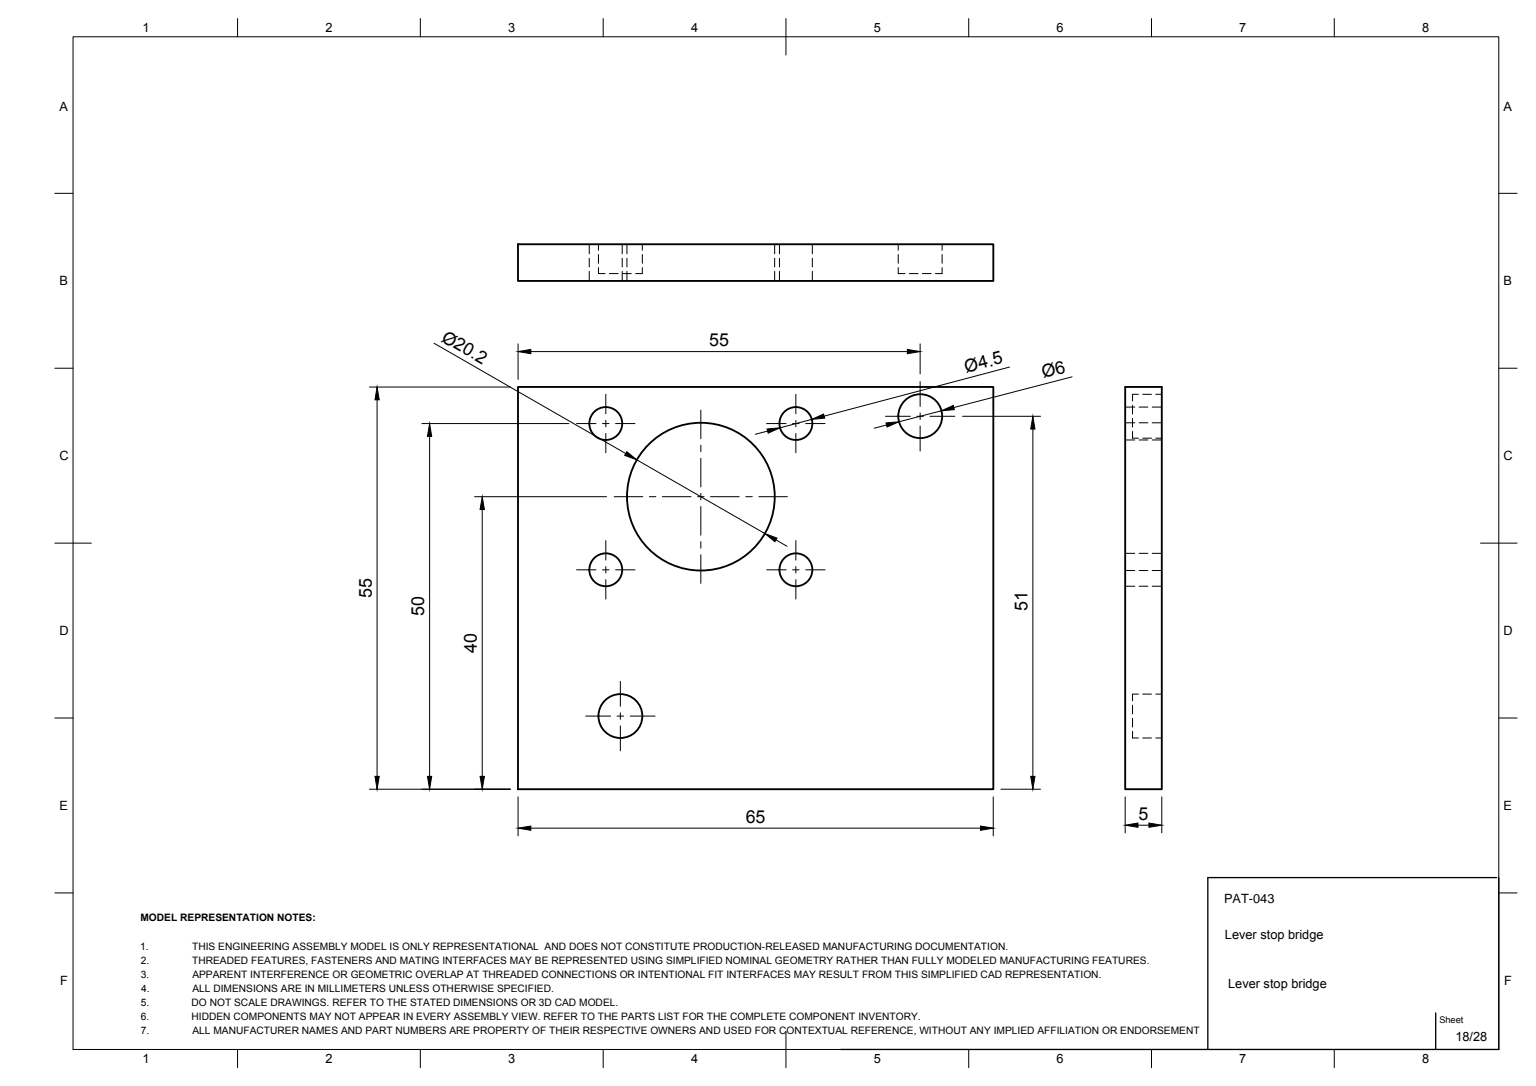
ISO-10303-21;
HEADER;
/* Generated by software containing ST-Developer
 * from STEP Tools, Inc. (www.steptools.com) 
 */

FILE_DESCRIPTION(
/* description */ ('Four-valve pipe header'),
/* implementation_level */ '2;1');

FILE_NAME(
/* name */ 'Lever stop bridge.step',
/* time_stamp */ '2026-10-29T16:56:19-07:00',
/* author */ (''),
/* organization */ (''),
/* preprocessor_version */ 'ST-DEVELOPER v20.2',
/* originating_system */ 'Autodesk Translation Framework v15.17.0.0',
/* authorisation */ '');

FILE_SCHEMA (('AUTOMOTIVE_DESIGN { 1 0 10303 214 3 1 1 }'));
ENDSEC;

DATA;
#10=MECHANICAL_DESIGN_GEOMETRIC_PRESENTATION_REPRESENTATION('',(#344),#10119);
#292=SHAPE_REPRESENTATION_RELATIONSHIP('SRR','None',#10254,#318);
#318=ADVANCED_BREP_SHAPE_REPRESENTATION('',(#370),#10103);
#344=STYLED_ITEM('',(#10456),#370);
#370=MANIFOLD_SOLID_BREP('Body1',#5590);
#498=FACE_BOUND('',#1339,.T.);
#499=FACE_BOUND('',#1340,.T.);
#500=FACE_BOUND('',#1341,.T.);
#501=FACE_BOUND('',#1342,.T.);
#502=FACE_BOUND('',#1343,.T.);
#503=FACE_BOUND('',#1344,.T.);
#504=FACE_BOUND('',#1345,.T.);
#505=FACE_BOUND('',#1347,.T.);
#506=FACE_BOUND('',#1348,.T.);
#507=FACE_BOUND('',#1349,.T.);
#508=FACE_BOUND('',#1350,.T.);
#509=FACE_BOUND('',#1351,.T.);
#636=PLANE('',#6253);
#637=PLANE('',#6257);
#638=PLANE('',#6273);
#639=PLANE('',#6274);
#640=PLANE('',#6275);
#641=PLANE('',#6276);
#642=PLANE('',#6277);
#643=PLANE('',#6278);
#921=FACE_OUTER_BOUND('',#1325,.T.);
#922=FACE_OUTER_BOUND('',#1326,.T.);
#923=FACE_OUTER_BOUND('',#1327,.T.);
#924=FACE_OUTER_BOUND('',#1328,.T.);
#925=FACE_OUTER_BOUND('',#1329,.T.);
#926=FACE_OUTER_BOUND('',#1330,.T.);
#927=FACE_OUTER_BOUND('',#1331,.T.);
#928=FACE_OUTER_BOUND('',#1332,.T.);
#929=FACE_OUTER_BOUND('',#1333,.T.);
#930=FACE_OUTER_BOUND('',#1334,.T.);
#931=FACE_OUTER_BOUND('',#1335,.T.);
#932=FACE_OUTER_BOUND('',#1336,.T.);
#933=FACE_OUTER_BOUND('',#1337,.T.);
#934=FACE_OUTER_BOUND('',#1338,.T.);
#935=FACE_OUTER_BOUND('',#1346,.T.);
#1325=EDGE_LOOP('',(#4523,#4524,#4525,#4526));
#1326=EDGE_LOOP('',(#4527));
#1327=EDGE_LOOP('',(#4528,#4529,#4530,#4531));
#1328=EDGE_LOOP('',(#4532));
#1329=EDGE_LOOP('',(#4533,#4534,#4535,#4536));
#1330=EDGE_LOOP('',(#4537,#4538,#4539,#4540));
#1331=EDGE_LOOP('',(#4541,#4542,#4543,#4544));
#1332=EDGE_LOOP('',(#4545,#4546,#4547,#4548));
#1333=EDGE_LOOP('',(#4549,#4550,#4551,#4552));
#1334=EDGE_LOOP('',(#4553,#4554,#4555,#4556));
#1335=EDGE_LOOP('',(#4557,#4558,#4559,#4560));
#1336=EDGE_LOOP('',(#4561,#4562,#4563,#4564));
#1337=EDGE_LOOP('',(#4565,#4566,#4567,#4568));
#1338=EDGE_LOOP('',(#4569,#4570,#4571,#4572));
#1339=EDGE_LOOP('',(#4573));
#1340=EDGE_LOOP('',(#4574));
#1341=EDGE_LOOP('',(#4575));
#1342=EDGE_LOOP('',(#4576));
#1343=EDGE_LOOP('',(#4577));
#1344=EDGE_LOOP('',(#4578));
#1345=EDGE_LOOP('',(#4579));
#1346=EDGE_LOOP('',(#4580,#4581,#4582,#4583));
#1347=EDGE_LOOP('',(#4584));
#1348=EDGE_LOOP('',(#4585));
#1349=EDGE_LOOP('',(#4586));
#1350=EDGE_LOOP('',(#4587));
#1351=EDGE_LOOP('',(#4588));
#1727=LINE('',#9294,#2145);
#1728=LINE('',#9301,#2146);
#1729=LINE('',#9308,#2147);
#1730=LINE('',#9314,#2148);
#1731=LINE('',#9320,#2149);
#1732=LINE('',#9326,#2150);
#1733=LINE('',#9332,#2151);
#1734=LINE('',#9337,#2152);
#1735=LINE('',#9339,#2153);
#1736=LINE('',#9341,#2154);
#1737=LINE('',#9342,#2155);
#1738=LINE('',#9345,#2156);
#1739=LINE('',#9347,#2157);
#1740=LINE('',#9348,#2158);
#1741=LINE('',#9351,#2159);
#1742=LINE('',#9353,#2160);
#1743=LINE('',#9354,#2161);
#1744=LINE('',#9356,#2162);
#1745=LINE('',#9357,#2163);
#2145=VECTOR('',#7490,0.3);
#2146=VECTOR('',#7499,0.3);
#2147=VECTOR('',#7508,0.225);
#2148=VECTOR('',#7515,0.225);
#2149=VECTOR('',#7522,0.225);
#2150=VECTOR('',#7529,0.225);
#2151=VECTOR('',#7536,1.01);
#2152=VECTOR('',#7541,1.);
#2153=VECTOR('',#7542,1.);
#2154=VECTOR('',#7543,1.);
#2155=VECTOR('',#7544,1.);
#2156=VECTOR('',#7547,1.);
#2157=VECTOR('',#7548,1.);
#2158=VECTOR('',#7549,1.);
#2159=VECTOR('',#7552,1.);
#2160=VECTOR('',#7553,1.);
#2161=VECTOR('',#7554,1.);
#2162=VECTOR('',#7557,1.);
#2163=VECTOR('',#7558,1.);
#2490=CIRCLE('',#6251,0.3);
#2491=CIRCLE('',#6252,0.3);
#2492=CIRCLE('',#6255,0.3);
#2493=CIRCLE('',#6256,0.3);
#2494=CIRCLE('',#6259,0.225);
#2495=CIRCLE('',#6260,0.225);
#2496=CIRCLE('',#6262,0.225);
#2497=CIRCLE('',#6263,0.225);
#2498=CIRCLE('',#6265,0.225);
#2499=CIRCLE('',#6266,0.225);
#2500=CIRCLE('',#6268,0.225);
#2501=CIRCLE('',#6269,0.225);
#2502=CIRCLE('',#6271,1.01);
#2503=CIRCLE('',#6272,1.01);
#2835=VERTEX_POINT('',#9291);
#2836=VERTEX_POINT('',#9293);
#2837=VERTEX_POINT('',#9298);
#2838=VERTEX_POINT('',#9300);
#2839=VERTEX_POINT('',#9305);
#2840=VERTEX_POINT('',#9307);
#2841=VERTEX_POINT('',#9311);
#2842=VERTEX_POINT('',#9313);
#2843=VERTEX_POINT('',#9317);
#2844=VERTEX_POINT('',#9319);
#2845=VERTEX_POINT('',#9323);
#2846=VERTEX_POINT('',#9325);
#2847=VERTEX_POINT('',#9329);
#2848=VERTEX_POINT('',#9331);
#2849=VERTEX_POINT('',#9335);
#2850=VERTEX_POINT('',#9336);
#2851=VERTEX_POINT('',#9338);
#2852=VERTEX_POINT('',#9340);
#2853=VERTEX_POINT('',#9344);
#2854=VERTEX_POINT('',#9346);
#2855=VERTEX_POINT('',#9350);
#2856=VERTEX_POINT('',#9352);
#3428=EDGE_CURVE('',#2835,#2835,#2490,.T.);
#3429=EDGE_CURVE('',#2835,#2836,#1727,.T.);
#3430=EDGE_CURVE('',#2836,#2836,#2491,.T.);
#3431=EDGE_CURVE('',#2837,#2837,#2492,.T.);
#3432=EDGE_CURVE('',#2837,#2838,#1728,.T.);
#3433=EDGE_CURVE('',#2838,#2838,#2493,.T.);
#3434=EDGE_CURVE('',#2839,#2839,#2494,.T.);
#3435=EDGE_CURVE('',#2839,#2840,#1729,.T.);
#3436=EDGE_CURVE('',#2840,#2840,#2495,.T.);
#3437=EDGE_CURVE('',#2841,#2841,#2496,.T.);
#3438=EDGE_CURVE('',#2841,#2842,#1730,.T.);
#3439=EDGE_CURVE('',#2842,#2842,#2497,.T.);
#3440=EDGE_CURVE('',#2843,#2843,#2498,.T.);
#3441=EDGE_CURVE('',#2843,#2844,#1731,.T.);
#3442=EDGE_CURVE('',#2844,#2844,#2499,.T.);
#3443=EDGE_CURVE('',#2845,#2845,#2500,.T.);
#3444=EDGE_CURVE('',#2845,#2846,#1732,.T.);
#3445=EDGE_CURVE('',#2846,#2846,#2501,.T.);
#3446=EDGE_CURVE('',#2847,#2847,#2502,.T.);
#3447=EDGE_CURVE('',#2847,#2848,#1733,.T.);
#3448=EDGE_CURVE('',#2848,#2848,#2503,.T.);
#3449=EDGE_CURVE('',#2849,#2850,#1734,.T.);
#3450=EDGE_CURVE('',#2850,#2851,#1735,.T.);
#3451=EDGE_CURVE('',#2852,#2851,#1736,.T.);
#3452=EDGE_CURVE('',#2849,#2852,#1737,.T.);
#3453=EDGE_CURVE('',#2853,#2849,#1738,.T.);
#3454=EDGE_CURVE('',#2854,#2852,#1739,.T.);
#3455=EDGE_CURVE('',#2853,#2854,#1740,.T.);
#3456=EDGE_CURVE('',#2855,#2853,#1741,.T.);
#3457=EDGE_CURVE('',#2856,#2854,#1742,.T.);
#3458=EDGE_CURVE('',#2855,#2856,#1743,.T.);
#3459=EDGE_CURVE('',#2850,#2855,#1744,.T.);
#3460=EDGE_CURVE('',#2851,#2856,#1745,.T.);
#4523=ORIENTED_EDGE('',*,*,#3428,.F.);
#4524=ORIENTED_EDGE('',*,*,#3429,.T.);
#4525=ORIENTED_EDGE('',*,*,#3430,.F.);
#4526=ORIENTED_EDGE('',*,*,#3429,.F.);
#4527=ORIENTED_EDGE('',*,*,#3428,.T.);
#4528=ORIENTED_EDGE('',*,*,#3431,.F.);
#4529=ORIENTED_EDGE('',*,*,#3432,.T.);
#4530=ORIENTED_EDGE('',*,*,#3433,.F.);
#4531=ORIENTED_EDGE('',*,*,#3432,.F.);
#4532=ORIENTED_EDGE('',*,*,#3431,.T.);
#4533=ORIENTED_EDGE('',*,*,#3434,.F.);
#4534=ORIENTED_EDGE('',*,*,#3435,.T.);
#4535=ORIENTED_EDGE('',*,*,#3436,.F.);
#4536=ORIENTED_EDGE('',*,*,#3435,.F.);
#4537=ORIENTED_EDGE('',*,*,#3437,.F.);
#4538=ORIENTED_EDGE('',*,*,#3438,.T.);
#4539=ORIENTED_EDGE('',*,*,#3439,.F.);
#4540=ORIENTED_EDGE('',*,*,#3438,.F.);
#4541=ORIENTED_EDGE('',*,*,#3440,.F.);
#4542=ORIENTED_EDGE('',*,*,#3441,.T.);
#4543=ORIENTED_EDGE('',*,*,#3442,.F.);
#4544=ORIENTED_EDGE('',*,*,#3441,.F.);
#4545=ORIENTED_EDGE('',*,*,#3443,.F.);
#4546=ORIENTED_EDGE('',*,*,#3444,.T.);
#4547=ORIENTED_EDGE('',*,*,#3445,.F.);
#4548=ORIENTED_EDGE('',*,*,#3444,.F.);
#4549=ORIENTED_EDGE('',*,*,#3446,.F.);
#4550=ORIENTED_EDGE('',*,*,#3447,.T.);
#4551=ORIENTED_EDGE('',*,*,#3448,.F.);
#4552=ORIENTED_EDGE('',*,*,#3447,.F.);
#4553=ORIENTED_EDGE('',*,*,#3449,.T.);
#4554=ORIENTED_EDGE('',*,*,#3450,.T.);
#4555=ORIENTED_EDGE('',*,*,#3451,.F.);
#4556=ORIENTED_EDGE('',*,*,#3452,.F.);
#4557=ORIENTED_EDGE('',*,*,#3453,.T.);
#4558=ORIENTED_EDGE('',*,*,#3452,.T.);
#4559=ORIENTED_EDGE('',*,*,#3454,.F.);
#4560=ORIENTED_EDGE('',*,*,#3455,.F.);
#4561=ORIENTED_EDGE('',*,*,#3456,.T.);
#4562=ORIENTED_EDGE('',*,*,#3455,.T.);
#4563=ORIENTED_EDGE('',*,*,#3457,.F.);
#4564=ORIENTED_EDGE('',*,*,#3458,.F.);
#4565=ORIENTED_EDGE('',*,*,#3459,.T.);
#4566=ORIENTED_EDGE('',*,*,#3458,.T.);
#4567=ORIENTED_EDGE('',*,*,#3460,.F.);
#4568=ORIENTED_EDGE('',*,*,#3450,.F.);
#4569=ORIENTED_EDGE('',*,*,#3460,.T.);
#4570=ORIENTED_EDGE('',*,*,#3457,.T.);
#4571=ORIENTED_EDGE('',*,*,#3454,.T.);
#4572=ORIENTED_EDGE('',*,*,#3451,.T.);
#4573=ORIENTED_EDGE('',*,*,#3430,.T.);
#4574=ORIENTED_EDGE('',*,*,#3433,.T.);
#4575=ORIENTED_EDGE('',*,*,#3448,.T.);
#4576=ORIENTED_EDGE('',*,*,#3445,.T.);
#4577=ORIENTED_EDGE('',*,*,#3442,.T.);
#4578=ORIENTED_EDGE('',*,*,#3439,.T.);
#4579=ORIENTED_EDGE('',*,*,#3436,.T.);
#4580=ORIENTED_EDGE('',*,*,#3459,.F.);
#4581=ORIENTED_EDGE('',*,*,#3449,.F.);
#4582=ORIENTED_EDGE('',*,*,#3453,.F.);
#4583=ORIENTED_EDGE('',*,*,#3456,.F.);
#4584=ORIENTED_EDGE('',*,*,#3446,.T.);
#4585=ORIENTED_EDGE('',*,*,#3443,.T.);
#4586=ORIENTED_EDGE('',*,*,#3440,.T.);
#4587=ORIENTED_EDGE('',*,*,#3437,.T.);
#4588=ORIENTED_EDGE('',*,*,#3434,.T.);
#5217=CYLINDRICAL_SURFACE('',#6250,0.3);
#5218=CYLINDRICAL_SURFACE('',#6254,0.3);
#5219=CYLINDRICAL_SURFACE('',#6258,0.225);
#5220=CYLINDRICAL_SURFACE('',#6261,0.225);
#5221=CYLINDRICAL_SURFACE('',#6264,0.225);
#5222=CYLINDRICAL_SURFACE('',#6267,0.225);
#5223=CYLINDRICAL_SURFACE('',#6270,1.01);
#5421=ADVANCED_FACE('',(#921),#5217,.F.);
#5422=ADVANCED_FACE('',(#922),#636,.T.);
#5423=ADVANCED_FACE('',(#923),#5218,.F.);
#5424=ADVANCED_FACE('',(#924),#637,.T.);
#5425=ADVANCED_FACE('',(#925),#5219,.F.);
#5426=ADVANCED_FACE('',(#926),#5220,.F.);
#5427=ADVANCED_FACE('',(#927),#5221,.F.);
#5428=ADVANCED_FACE('',(#928),#5222,.F.);
#5429=ADVANCED_FACE('',(#929),#5223,.F.);
#5430=ADVANCED_FACE('',(#930),#638,.T.);
#5431=ADVANCED_FACE('',(#931),#639,.T.);
#5432=ADVANCED_FACE('',(#932),#640,.T.);
#5433=ADVANCED_FACE('',(#933),#641,.T.);
#5434=ADVANCED_FACE('',(#934,#498,#499,#500,#501,#502,#503,#504),#642,.T.);
#5435=ADVANCED_FACE('',(#935,#505,#506,#507,#508,#509),#643,.F.);
#5590=CLOSED_SHELL('',(#5421,#5422,#5423,#5424,#5425,#5426,#5427,#5428,
#5429,#5430,#5431,#5432,#5433,#5434,#5435));
#6249=AXIS2_PLACEMENT_3D('',#9289,#7484,#7485);
#6250=AXIS2_PLACEMENT_3D('',#9290,#7486,#7487);
#6251=AXIS2_PLACEMENT_3D('',#9292,#7488,#7489);
#6252=AXIS2_PLACEMENT_3D('',#9295,#7491,#7492);
#6253=AXIS2_PLACEMENT_3D('',#9296,#7493,#7494);
#6254=AXIS2_PLACEMENT_3D('',#9297,#7495,#7496);
#6255=AXIS2_PLACEMENT_3D('',#9299,#7497,#7498);
#6256=AXIS2_PLACEMENT_3D('',#9302,#7500,#7501);
#6257=AXIS2_PLACEMENT_3D('',#9303,#7502,#7503);
#6258=AXIS2_PLACEMENT_3D('',#9304,#7504,#7505);
#6259=AXIS2_PLACEMENT_3D('',#9306,#7506,#7507);
#6260=AXIS2_PLACEMENT_3D('',#9309,#7509,#7510);
#6261=AXIS2_PLACEMENT_3D('',#9310,#7511,#7512);
#6262=AXIS2_PLACEMENT_3D('',#9312,#7513,#7514);
#6263=AXIS2_PLACEMENT_3D('',#9315,#7516,#7517);
#6264=AXIS2_PLACEMENT_3D('',#9316,#7518,#7519);
#6265=AXIS2_PLACEMENT_3D('',#9318,#7520,#7521);
#6266=AXIS2_PLACEMENT_3D('',#9321,#7523,#7524);
#6267=AXIS2_PLACEMENT_3D('',#9322,#7525,#7526);
#6268=AXIS2_PLACEMENT_3D('',#9324,#7527,#7528);
#6269=AXIS2_PLACEMENT_3D('',#9327,#7530,#7531);
#6270=AXIS2_PLACEMENT_3D('',#9328,#7532,#7533);
#6271=AXIS2_PLACEMENT_3D('',#9330,#7534,#7535);
#6272=AXIS2_PLACEMENT_3D('',#9333,#7537,#7538);
#6273=AXIS2_PLACEMENT_3D('',#9334,#7539,#7540);
#6274=AXIS2_PLACEMENT_3D('',#9343,#7545,#7546);
#6275=AXIS2_PLACEMENT_3D('',#9349,#7550,#7551);
#6276=AXIS2_PLACEMENT_3D('',#9355,#7555,#7556);
#6277=AXIS2_PLACEMENT_3D('',#9358,#7559,#7560);
#6278=AXIS2_PLACEMENT_3D('',#9359,#7561,#7562);
#7484=DIRECTION('axis',(0.,0.,1.));
#7485=DIRECTION('refdir',(1.,0.,0.));
#7486=DIRECTION('center_axis',(0.,0.,1.));
#7487=DIRECTION('ref_axis',(1.,0.,0.));
#7488=DIRECTION('center_axis',(0.,0.,1.));
#7489=DIRECTION('ref_axis',(1.,0.,0.));
#7490=DIRECTION('',(0.,0.,1.));
#7491=DIRECTION('center_axis',(0.,0.,-1.));
#7492=DIRECTION('ref_axis',(1.,0.,0.));
#7493=DIRECTION('center_axis',(0.,0.,1.));
#7494=DIRECTION('ref_axis',(1.,0.,0.));
#7495=DIRECTION('center_axis',(0.,0.,1.));
#7496=DIRECTION('ref_axis',(1.,0.,0.));
#7497=DIRECTION('center_axis',(0.,0.,1.));
#7498=DIRECTION('ref_axis',(1.,0.,0.));
#7499=DIRECTION('',(0.,0.,1.));
#7500=DIRECTION('center_axis',(0.,0.,-1.));
#7501=DIRECTION('ref_axis',(1.,0.,0.));
#7502=DIRECTION('center_axis',(0.,0.,1.));
#7503=DIRECTION('ref_axis',(1.,0.,0.));
#7504=DIRECTION('center_axis',(0.,0.,1.));
#7505=DIRECTION('ref_axis',(1.,0.,0.));
#7506=DIRECTION('center_axis',(0.,0.,1.));
#7507=DIRECTION('ref_axis',(1.,0.,0.));
#7508=DIRECTION('',(0.,0.,1.));
#7509=DIRECTION('center_axis',(0.,0.,-1.));
#7510=DIRECTION('ref_axis',(1.,0.,0.));
#7511=DIRECTION('center_axis',(0.,0.,1.));
#7512=DIRECTION('ref_axis',(1.,0.,0.));
#7513=DIRECTION('center_axis',(0.,0.,1.));
#7514=DIRECTION('ref_axis',(1.,0.,0.));
#7515=DIRECTION('',(0.,0.,1.));
#7516=DIRECTION('center_axis',(0.,0.,-1.));
#7517=DIRECTION('ref_axis',(1.,0.,0.));
#7518=DIRECTION('center_axis',(0.,0.,1.));
#7519=DIRECTION('ref_axis',(1.,0.,0.));
#7520=DIRECTION('center_axis',(0.,0.,1.));
#7521=DIRECTION('ref_axis',(1.,0.,0.));
#7522=DIRECTION('',(0.,0.,1.));
#7523=DIRECTION('center_axis',(0.,0.,-1.));
#7524=DIRECTION('ref_axis',(1.,0.,0.));
#7525=DIRECTION('center_axis',(0.,0.,1.));
#7526=DIRECTION('ref_axis',(1.,0.,0.));
#7527=DIRECTION('center_axis',(0.,0.,1.));
#7528=DIRECTION('ref_axis',(1.,0.,0.));
#7529=DIRECTION('',(0.,0.,1.));
#7530=DIRECTION('center_axis',(0.,0.,-1.));
#7531=DIRECTION('ref_axis',(1.,0.,0.));
#7532=DIRECTION('center_axis',(0.,0.,1.));
#7533=DIRECTION('ref_axis',(1.,0.,0.));
#7534=DIRECTION('center_axis',(0.,0.,1.));
#7535=DIRECTION('ref_axis',(1.,0.,0.));
#7536=DIRECTION('',(0.,0.,1.));
#7537=DIRECTION('center_axis',(0.,0.,-1.));
#7538=DIRECTION('ref_axis',(1.,0.,0.));
#7539=DIRECTION('center_axis',(0.,1.,0.));
#7540=DIRECTION('ref_axis',(-1.,0.,0.));
#7541=DIRECTION('',(-1.,0.,0.));
#7542=DIRECTION('',(0.,0.,1.));
#7543=DIRECTION('',(-1.,0.,0.));
#7544=DIRECTION('',(0.,0.,1.));
#7545=DIRECTION('center_axis',(1.,0.,0.));
#7546=DIRECTION('ref_axis',(0.,1.,0.));
#7547=DIRECTION('',(0.,1.,0.));
#7548=DIRECTION('',(0.,1.,0.));
#7549=DIRECTION('',(0.,0.,1.));
#7550=DIRECTION('center_axis',(0.,-1.,0.));
#7551=DIRECTION('ref_axis',(1.,0.,0.));
#7552=DIRECTION('',(1.,0.,0.));
#7553=DIRECTION('',(1.,0.,0.));
#7554=DIRECTION('',(0.,0.,1.));
#7555=DIRECTION('center_axis',(-1.,0.,0.));
#7556=DIRECTION('ref_axis',(0.,-1.,0.));
#7557=DIRECTION('',(0.,-1.,0.));
#7558=DIRECTION('',(0.,-1.,0.));
#7559=DIRECTION('center_axis',(0.,0.,1.));
#7560=DIRECTION('ref_axis',(1.,0.,0.));
#7561=DIRECTION('center_axis',(0.,0.,1.));
#7562=DIRECTION('ref_axis',(1.,0.,0.));
#9289=CARTESIAN_POINT('',(0.,0.,0.));
#9290=CARTESIAN_POINT('Origin',(-1.1,-3.,8.1));
#9291=CARTESIAN_POINT('',(-1.4,-3.,8.1));
#9292=CARTESIAN_POINT('Origin',(-1.1,-3.,8.1));
#9293=CARTESIAN_POINT('',(-1.4,-3.,8.5));
#9294=CARTESIAN_POINT('',(-1.4,-3.,8.1));
#9295=CARTESIAN_POINT('Origin',(-1.1,-3.,8.5));
#9296=CARTESIAN_POINT('Origin',(-1.1,-3.,8.1));
#9297=CARTESIAN_POINT('Origin',(3.,1.1,8.1));
#9298=CARTESIAN_POINT('',(2.7,1.1,8.1));
#9299=CARTESIAN_POINT('Origin',(3.,1.1,8.1));
#9300=CARTESIAN_POINT('',(2.7,1.1,8.5));
#9301=CARTESIAN_POINT('',(2.7,1.1,8.1));
#9302=CARTESIAN_POINT('Origin',(3.,1.1,8.5));
#9303=CARTESIAN_POINT('Origin',(3.,1.1,8.1));
#9304=CARTESIAN_POINT('Origin',(1.3,-1.,7.9));
#9305=CARTESIAN_POINT('',(1.075,-1.,8.));
#9306=CARTESIAN_POINT('Origin',(1.3,-1.,8.));
#9307=CARTESIAN_POINT('',(1.075,-1.,8.5));
#9308=CARTESIAN_POINT('',(1.075,-1.,7.9));
#9309=CARTESIAN_POINT('Origin',(1.3,-1.,8.5));
#9310=CARTESIAN_POINT('Origin',(-1.3,1.,7.9));
#9311=CARTESIAN_POINT('',(-1.525,1.,8.));
#9312=CARTESIAN_POINT('Origin',(-1.3,1.,8.));
#9313=CARTESIAN_POINT('',(-1.525,1.,8.5));
#9314=CARTESIAN_POINT('',(-1.525,1.,7.9));
#9315=CARTESIAN_POINT('Origin',(-1.3,1.,8.5));
#9316=CARTESIAN_POINT('Origin',(-1.3,-1.,7.9));
#9317=CARTESIAN_POINT('',(-1.525,-1.,8.));
#9318=CARTESIAN_POINT('Origin',(-1.3,-1.,8.));
#9319=CARTESIAN_POINT('',(-1.525,-1.,8.5));
#9320=CARTESIAN_POINT('',(-1.525,-1.,7.9));
#9321=CARTESIAN_POINT('Origin',(-1.3,-1.,8.5));
#9322=CARTESIAN_POINT('Origin',(1.3,1.,7.9));
#9323=CARTESIAN_POINT('',(1.075,1.,8.));
#9324=CARTESIAN_POINT('Origin',(1.3,1.,8.));
#9325=CARTESIAN_POINT('',(1.075,1.,8.5));
#9326=CARTESIAN_POINT('',(1.075,1.,7.9));
#9327=CARTESIAN_POINT('Origin',(1.3,1.,8.5));
#9328=CARTESIAN_POINT('Origin',(0.,0.,7.9));
#9329=CARTESIAN_POINT('',(-1.01,-1.23689326713883E-16,8.));
#9330=CARTESIAN_POINT('Origin',(0.,0.,8.));
#9331=CARTESIAN_POINT('',(-1.01,1.23689326713883E-16,8.5));
#9332=CARTESIAN_POINT('',(-1.01,-1.23689326713883E-16,7.9));
#9333=CARTESIAN_POINT('Origin',(0.,0.,8.5));
#9334=CARTESIAN_POINT('Origin',(4.,1.5,8.));
#9335=CARTESIAN_POINT('',(4.,1.5,8.));
#9336=CARTESIAN_POINT('',(-2.5,1.5,8.));
#9337=CARTESIAN_POINT('',(4.,1.5,8.));
#9338=CARTESIAN_POINT('',(-2.5,1.5,8.5));
#9339=CARTESIAN_POINT('',(-2.5,1.5,8.));
#9340=CARTESIAN_POINT('',(4.,1.5,8.5));
#9341=CARTESIAN_POINT('',(4.,1.5,8.5));
#9342=CARTESIAN_POINT('',(4.,1.5,8.));
#9343=CARTESIAN_POINT('Origin',(4.,-4.,8.));
#9344=CARTESIAN_POINT('',(4.,-4.,8.));
#9345=CARTESIAN_POINT('',(4.,-4.,8.));
#9346=CARTESIAN_POINT('',(4.,-4.,8.5));
#9347=CARTESIAN_POINT('',(4.,-4.,8.5));
#9348=CARTESIAN_POINT('',(4.,-4.,8.));
#9349=CARTESIAN_POINT('Origin',(-2.5,-4.,8.));
#9350=CARTESIAN_POINT('',(-2.5,-4.,8.));
#9351=CARTESIAN_POINT('',(-2.5,-4.,8.));
#9352=CARTESIAN_POINT('',(-2.5,-4.,8.5));
#9353=CARTESIAN_POINT('',(-2.5,-4.,8.5));
#9354=CARTESIAN_POINT('',(-2.5,-4.,8.));
#9355=CARTESIAN_POINT('Origin',(-2.5,1.5,8.));
#9356=CARTESIAN_POINT('',(-2.5,1.5,8.));
#9357=CARTESIAN_POINT('',(-2.5,1.5,8.5));
#9358=CARTESIAN_POINT('Origin',(0.75,-1.25,8.5));
#9359=CARTESIAN_POINT('Origin',(0.75,-1.25,8.));
#10072=UNCERTAINTY_MEASURE_WITH_UNIT(LENGTH_MEASURE(0.001),#10120,
'DISTANCE_ACCURACY_VALUE',
'Maximum model space distance between geometric entities at asserted c
onnectivities');
#10088=UNCERTAINTY_MEASURE_WITH_UNIT(LENGTH_MEASURE(0.001),#10120,
'DISTANCE_ACCURACY_VALUE',
'Maximum model space distance between geometric entities at asserted c
onnectivities');
#10103=(
GEOMETRIC_REPRESENTATION_CONTEXT(3)
GLOBAL_UNCERTAINTY_ASSIGNED_CONTEXT((#10072))
GLOBAL_UNIT_ASSIGNED_CONTEXT((#10120,#10122,#10123))
REPRESENTATION_CONTEXT('','3D')
);
#10119=(
GEOMETRIC_REPRESENTATION_CONTEXT(3)
GLOBAL_UNCERTAINTY_ASSIGNED_CONTEXT((#10088))
GLOBAL_UNIT_ASSIGNED_CONTEXT((#10120,#10122,#10123))
REPRESENTATION_CONTEXT('','3D')
);
#10120=(
LENGTH_UNIT()
NAMED_UNIT(*)
SI_UNIT(.CENTI.,.METRE.)
);
#10122=(
NAMED_UNIT(*)
PLANE_ANGLE_UNIT()
SI_UNIT($,.RADIAN.)
);
#10123=(
NAMED_UNIT(*)
SI_UNIT($,.STERADIAN.)
SOLID_ANGLE_UNIT()
);
#10138=SHAPE_DEFINITION_REPRESENTATION(#10168,#10254);
#10168=PRODUCT_DEFINITION_SHAPE('',$,#10285);
#10254=SHAPE_REPRESENTATION('',(#6249),#10103);
#10270=PRODUCT_DEFINITION_CONTEXT('part definition',#10362,'design');
#10285=PRODUCT_DEFINITION('Lever stop bridge','Lever stop bridge',#10315,
#10270);
#10315=PRODUCT_DEFINITION_FORMATION('',$,#10378);
#10362=APPLICATION_CONTEXT(
'Core Data for Automotive Mechanical Design Process');
#10363=PRODUCT_CONTEXT('part definition',#10362,'mechanical');
#10378=PRODUCT('Lever stop bridge','Lever stop bridge',
'Lever stop bridge',(#10363));
#10450=COLOUR_RGB('Light Blue',0.38,0.62,0.78);
#10451=FILL_AREA_STYLE_COLOUR('',#10450);
#10452=FILL_AREA_STYLE('',(#10451));
#10453=SURFACE_STYLE_FILL_AREA(#10452);
#10454=SURFACE_SIDE_STYLE('',(#10453));
#10455=SURFACE_STYLE_USAGE(.BOTH.,#10454);
#10456=PRESENTATION_STYLE_ASSIGNMENT((#10455));
ENDSEC;
END-ISO-10303-21;
